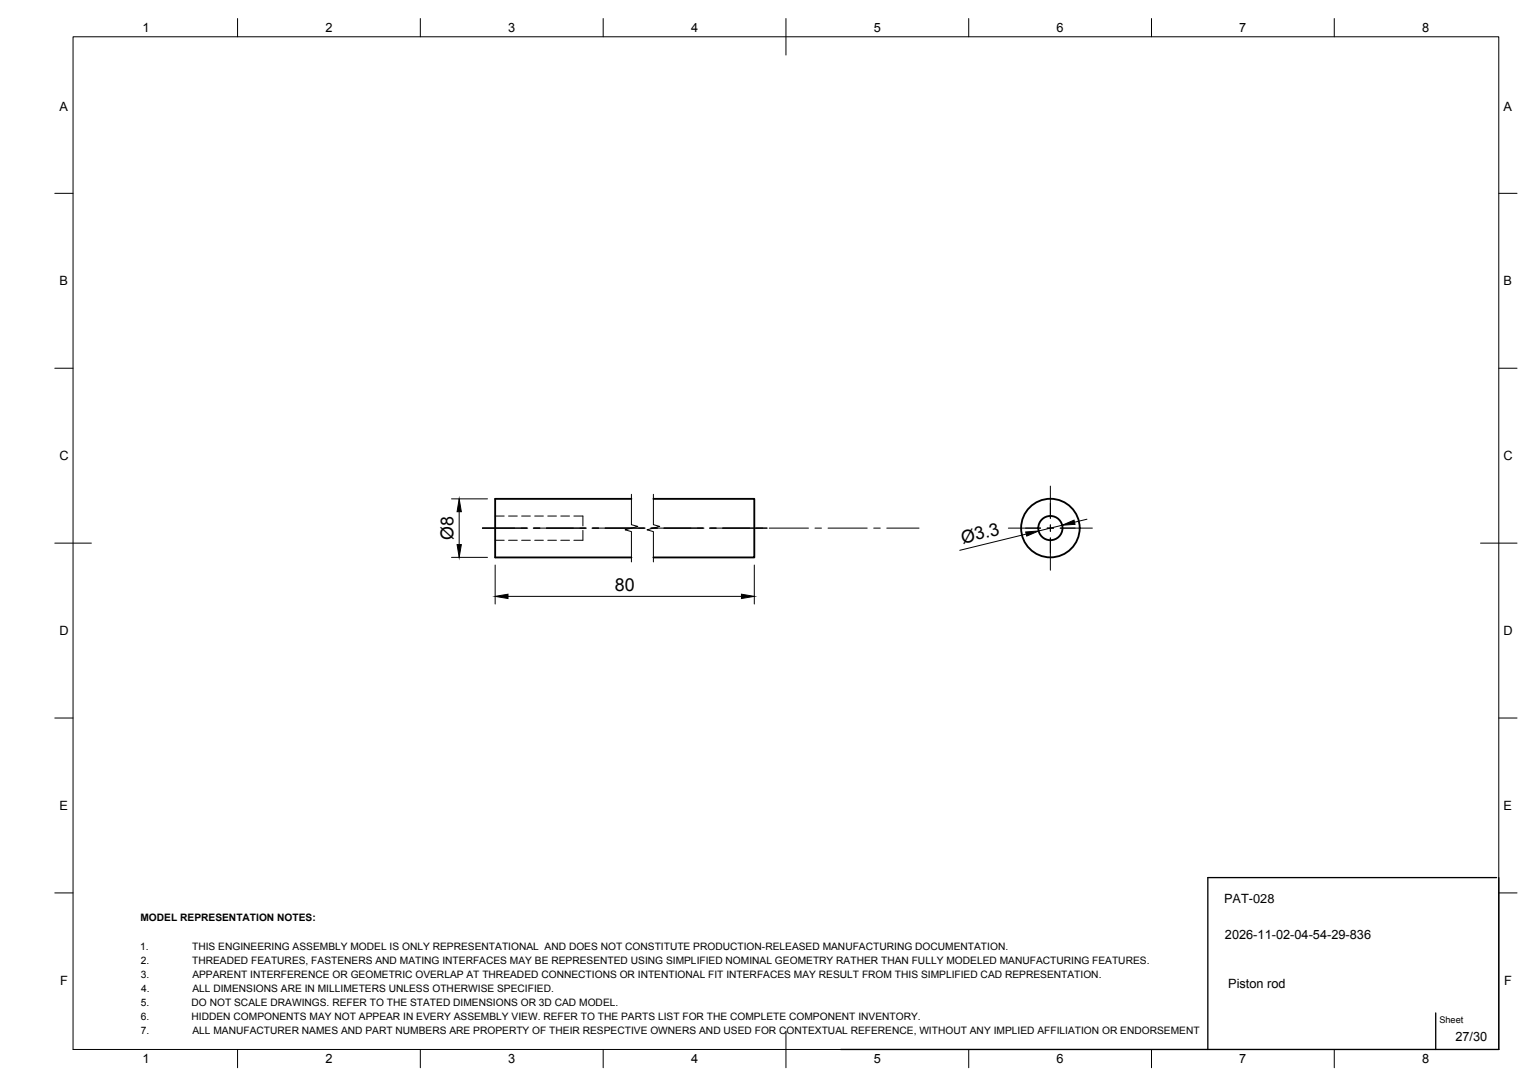
ISO-10303-21;
HEADER;
/* Generated by software containing ST-Developer
 * from STEP Tools, Inc. (www.steptools.com) 
 */

FILE_DESCRIPTION(
/* description */ ('Cylinder foot and clevis mount kit'),
/* implementation_level */ '2;1');

FILE_NAME(
/* name */ 'Piston rod.step',
/* time_stamp */ '2026-10-27T20:10:43-07:00',
/* author */ (''),
/* organization */ (''),
/* preprocessor_version */ 'ST-DEVELOPER v20.2',
/* originating_system */ 'Autodesk Translation Framework v15.17.0.0',
/* authorisation */ '');

FILE_SCHEMA (('AUTOMOTIVE_DESIGN { 1 0 10303 214 3 1 1 }'));
ENDSEC;

DATA;
#10=MECHANICAL_DESIGN_GEOMETRIC_PRESENTATION_REPRESENTATION('',(#359),#9102);
#303=SHAPE_REPRESENTATION_RELATIONSHIP('SRR','None',#9252,#331);
#331=ADVANCED_BREP_SHAPE_REPRESENTATION('',(#386),#9095);
#359=STYLED_ITEM('',(#9460),#386);
#386=MANIFOLD_SOLID_BREP('Body1',#4946);
#479=FACE_BOUND('',#1331,.T.);
#652=PLANE('',#5767);
#653=PLANE('',#5771);
#654=PLANE('',#5772);
#934=FACE_OUTER_BOUND('',#1327,.T.);
#935=FACE_OUTER_BOUND('',#1328,.T.);
#936=FACE_OUTER_BOUND('',#1329,.T.);
#937=FACE_OUTER_BOUND('',#1330,.T.);
#938=FACE_OUTER_BOUND('',#1332,.T.);
#1327=EDGE_LOOP('',(#4243,#4244,#4245,#4246));
#1328=EDGE_LOOP('',(#4247));
#1329=EDGE_LOOP('',(#4248,#4249,#4250,#4251));
#1330=EDGE_LOOP('',(#4252));
#1331=EDGE_LOOP('',(#4253));
#1332=EDGE_LOOP('',(#4254));
#1669=LINE('',#8590,#2018);
#1670=LINE('',#8597,#2019);
#2018=VECTOR('',#7156,0.165);
#2019=VECTOR('',#7165,0.4);
#2287=CIRCLE('',#5765,0.165);
#2288=CIRCLE('',#5766,0.165);
#2289=CIRCLE('',#5769,0.4);
#2290=CIRCLE('',#5770,0.4);
#2622=VERTEX_POINT('',#8587);
#2623=VERTEX_POINT('',#8589);
#2624=VERTEX_POINT('',#8594);
#2625=VERTEX_POINT('',#8596);
#3176=EDGE_CURVE('',#2622,#2622,#2287,.T.);
#3177=EDGE_CURVE('',#2622,#2623,#1669,.T.);
#3178=EDGE_CURVE('',#2623,#2623,#2288,.T.);
#3179=EDGE_CURVE('',#2624,#2624,#2289,.T.);
#3180=EDGE_CURVE('',#2624,#2625,#1670,.T.);
#3181=EDGE_CURVE('',#2625,#2625,#2290,.T.);
#4243=ORIENTED_EDGE('',*,*,#3176,.F.);
#4244=ORIENTED_EDGE('',*,*,#3177,.T.);
#4245=ORIENTED_EDGE('',*,*,#3178,.F.);
#4246=ORIENTED_EDGE('',*,*,#3177,.F.);
#4247=ORIENTED_EDGE('',*,*,#3176,.T.);
#4248=ORIENTED_EDGE('',*,*,#3179,.F.);
#4249=ORIENTED_EDGE('',*,*,#3180,.T.);
#4250=ORIENTED_EDGE('',*,*,#3181,.T.);
#4251=ORIENTED_EDGE('',*,*,#3180,.F.);
#4252=ORIENTED_EDGE('',*,*,#3179,.T.);
#4253=ORIENTED_EDGE('',*,*,#3178,.T.);
#4254=ORIENTED_EDGE('',*,*,#3181,.F.);
#4603=CYLINDRICAL_SURFACE('',#5764,0.165);
#4604=CYLINDRICAL_SURFACE('',#5768,0.4);
#4857=ADVANCED_FACE('',(#934),#4603,.F.);
#4858=ADVANCED_FACE('',(#935),#652,.T.);
#4859=ADVANCED_FACE('',(#936),#4604,.T.);
#4860=ADVANCED_FACE('',(#937,#479),#653,.T.);
#4861=ADVANCED_FACE('',(#938),#654,.F.);
#4946=CLOSED_SHELL('',(#4857,#4858,#4859,#4860,#4861));
#5763=AXIS2_PLACEMENT_3D('',#8585,#7150,#7151);
#5764=AXIS2_PLACEMENT_3D('',#8586,#7152,#7153);
#5765=AXIS2_PLACEMENT_3D('',#8588,#7154,#7155);
#5766=AXIS2_PLACEMENT_3D('',#8591,#7157,#7158);
#5767=AXIS2_PLACEMENT_3D('',#8592,#7159,#7160);
#5768=AXIS2_PLACEMENT_3D('',#8593,#7161,#7162);
#5769=AXIS2_PLACEMENT_3D('',#8595,#7163,#7164);
#5770=AXIS2_PLACEMENT_3D('',#8598,#7166,#7167);
#5771=AXIS2_PLACEMENT_3D('',#8599,#7168,#7169);
#5772=AXIS2_PLACEMENT_3D('',#8600,#7170,#7171);
#7150=DIRECTION('axis',(0.,0.,1.));
#7151=DIRECTION('refdir',(1.,0.,0.));
#7152=DIRECTION('center_axis',(0.,1.,0.));
#7153=DIRECTION('ref_axis',(1.,0.,0.));
#7154=DIRECTION('center_axis',(0.,1.,0.));
#7155=DIRECTION('ref_axis',(1.,0.,0.));
#7156=DIRECTION('',(0.,1.,0.));
#7157=DIRECTION('center_axis',(0.,-1.,0.));
#7158=DIRECTION('ref_axis',(1.,0.,0.));
#7159=DIRECTION('center_axis',(0.,1.,0.));
#7160=DIRECTION('ref_axis',(1.,0.,0.));
#7161=DIRECTION('center_axis',(0.,1.,0.));
#7162=DIRECTION('ref_axis',(1.,0.,0.));
#7163=DIRECTION('center_axis',(0.,1.,0.));
#7164=DIRECTION('ref_axis',(1.,0.,0.));
#7165=DIRECTION('',(0.,-1.,0.));
#7166=DIRECTION('center_axis',(0.,1.,0.));
#7167=DIRECTION('ref_axis',(1.,0.,0.));
#7168=DIRECTION('center_axis',(0.,1.,0.));
#7169=DIRECTION('ref_axis',(1.,0.,0.));
#7170=DIRECTION('center_axis',(0.,1.,0.));
#7171=DIRECTION('ref_axis',(1.,0.,0.));
#8585=CARTESIAN_POINT('',(0.,0.,0.));
#8586=CARTESIAN_POINT('Origin',(0.,1.2,4.5));
#8587=CARTESIAN_POINT('',(-0.165,1.2,4.5));
#8588=CARTESIAN_POINT('Origin',(0.,1.2,4.5));
#8589=CARTESIAN_POINT('',(-0.165,2.4,4.5));
#8590=CARTESIAN_POINT('',(-0.165,1.2,4.5));
#8591=CARTESIAN_POINT('Origin',(0.,2.4,4.5));
#8592=CARTESIAN_POINT('Origin',(0.,1.2,4.5));
#8593=CARTESIAN_POINT('Origin',(0.,-5.6,4.5));
#8594=CARTESIAN_POINT('',(-0.4,2.4,4.5));
#8595=CARTESIAN_POINT('Origin',(0.,2.4,4.5));
#8596=CARTESIAN_POINT('',(-0.4,-5.6,4.5));
#8597=CARTESIAN_POINT('',(-0.4,-5.6,4.5));
#8598=CARTESIAN_POINT('Origin',(0.,-5.6,4.5));
#8599=CARTESIAN_POINT('Origin',(0.,2.4,4.5));
#8600=CARTESIAN_POINT('Origin',(0.,-5.6,4.5));
#9062=UNCERTAINTY_MEASURE_WITH_UNIT(LENGTH_MEASURE(0.001),#9103,
'DISTANCE_ACCURACY_VALUE',
'Maximum model space distance between geometric entities at asserted c
onnectivities');
#9069=UNCERTAINTY_MEASURE_WITH_UNIT(LENGTH_MEASURE(0.001),#9103,
'DISTANCE_ACCURACY_VALUE',
'Maximum model space distance between geometric entities at asserted c
onnectivities');
#9095=(
GEOMETRIC_REPRESENTATION_CONTEXT(3)
GLOBAL_UNCERTAINTY_ASSIGNED_CONTEXT((#9062))
GLOBAL_UNIT_ASSIGNED_CONTEXT((#9103,#9105,#9106))
REPRESENTATION_CONTEXT('','3D')
);
#9102=(
GEOMETRIC_REPRESENTATION_CONTEXT(3)
GLOBAL_UNCERTAINTY_ASSIGNED_CONTEXT((#9069))
GLOBAL_UNIT_ASSIGNED_CONTEXT((#9103,#9105,#9106))
REPRESENTATION_CONTEXT('','3D')
);
#9103=(
LENGTH_UNIT()
NAMED_UNIT(*)
SI_UNIT(.CENTI.,.METRE.)
);
#9105=(
NAMED_UNIT(*)
PLANE_ANGLE_UNIT()
SI_UNIT($,.RADIAN.)
);
#9106=(
NAMED_UNIT(*)
SI_UNIT($,.STERADIAN.)
SOLID_ANGLE_UNIT()
);
#9132=SHAPE_DEFINITION_REPRESENTATION(#9207,#9252);
#9207=PRODUCT_DEFINITION_SHAPE('',$,#9285);
#9252=SHAPE_REPRESENTATION('',(#5763),#9095);
#9259=PRODUCT_DEFINITION_CONTEXT('part definition',#9357,'design');
#9285=PRODUCT_DEFINITION('Piston rod','Piston rod',#9317,#9259);
#9317=PRODUCT_DEFINITION_FORMATION('',$,#9384);
#9357=APPLICATION_CONTEXT(
'Core Data for Automotive Mechanical Design Process');
#9358=PRODUCT_CONTEXT('part definition',#9357,'mechanical');
#9384=PRODUCT('Piston rod','Piston rod','Piston rod',(#9358));
#9454=COLOUR_RGB('Grey',0.48,0.52,0.57);
#9455=FILL_AREA_STYLE_COLOUR('',#9454);
#9456=FILL_AREA_STYLE('',(#9455));
#9457=SURFACE_STYLE_FILL_AREA(#9456);
#9458=SURFACE_SIDE_STYLE('',(#9457));
#9459=SURFACE_STYLE_USAGE(.BOTH.,#9458);
#9460=PRESENTATION_STYLE_ASSIGNMENT((#9459));
ENDSEC;
END-ISO-10303-21;
